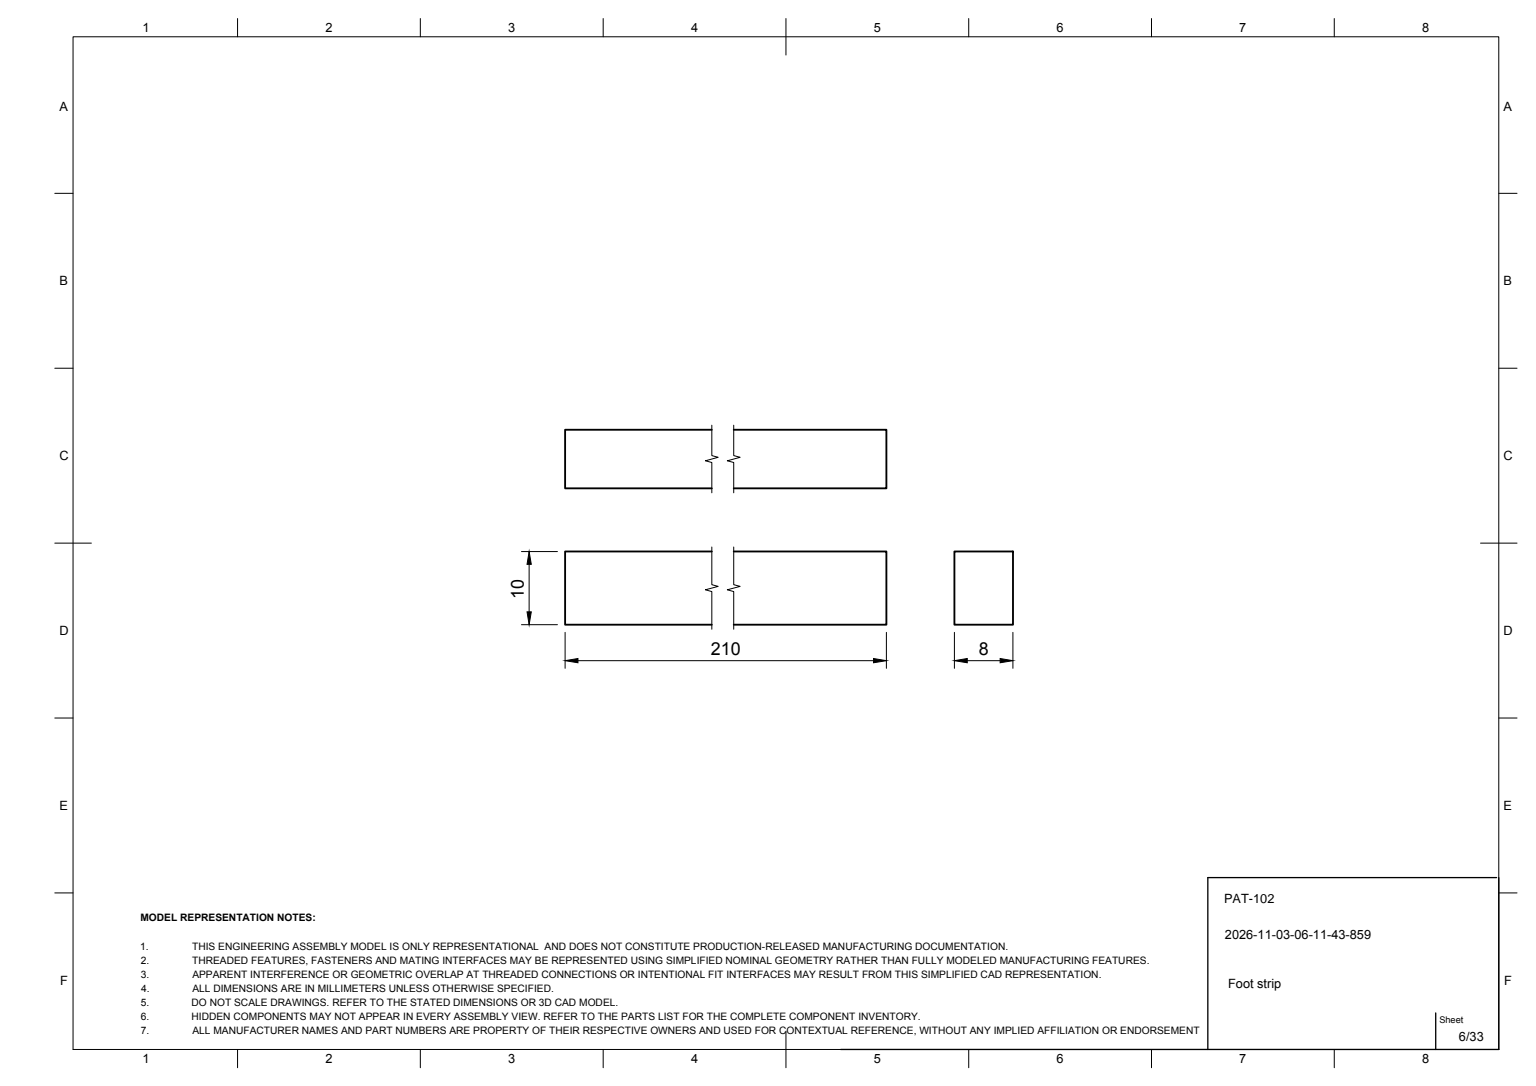
ISO-10303-21;
HEADER;
/* Generated by software containing ST-Developer
 * from STEP Tools, Inc. (www.steptools.com) 
 */

FILE_DESCRIPTION(
/* description */ ('Swing-away clamp arm'),
/* implementation_level */ '2;1');

FILE_NAME(
/* name */ 'Foot strip.step',
/* time_stamp */ '2026-10-28T03:26:03-07:00',
/* author */ (''),
/* organization */ (''),
/* preprocessor_version */ 'ST-DEVELOPER v20.2',
/* originating_system */ 'Autodesk Translation Framework v15.17.0.0',
/* authorisation */ '');

FILE_SCHEMA (('AUTOMOTIVE_DESIGN { 1 0 10303 214 3 1 1 }'));
ENDSEC;

DATA;
#10=MECHANICAL_DESIGN_GEOMETRIC_PRESENTATION_REPRESENTATION('',(#294),#10627);
#242=SHAPE_REPRESENTATION_RELATIONSHIP('SRR','None',#10740,#268);
#268=ADVANCED_BREP_SHAPE_REPRESENTATION('',(#328),#10599);
#294=STYLED_ITEM('',(#10951),#328);
#328=MANIFOLD_SOLID_BREP('Body1',#4900);
#464=PLANE('',#5245);
#465=PLANE('',#5246);
#466=PLANE('',#5247);
#467=PLANE('',#5248);
#468=PLANE('',#5249);
#469=PLANE('',#5250);
#647=FACE_OUTER_BOUND('',#962,.T.);
#648=FACE_OUTER_BOUND('',#963,.T.);
#649=FACE_OUTER_BOUND('',#964,.T.);
#650=FACE_OUTER_BOUND('',#965,.T.);
#651=FACE_OUTER_BOUND('',#966,.T.);
#652=FACE_OUTER_BOUND('',#967,.T.);
#962=EDGE_LOOP('',(#3329,#3330,#3331,#3332));
#963=EDGE_LOOP('',(#3333,#3334,#3335,#3336));
#964=EDGE_LOOP('',(#3337,#3338,#3339,#3340));
#965=EDGE_LOOP('',(#3341,#3342,#3343,#3344));
#966=EDGE_LOOP('',(#3345,#3346,#3347,#3348));
#967=EDGE_LOOP('',(#3349,#3350,#3351,#3352));
#1367=LINE('',#7543,#1689);
#1368=LINE('',#7545,#1690);
#1369=LINE('',#7547,#1691);
#1370=LINE('',#7548,#1692);
#1371=LINE('',#7551,#1693);
#1372=LINE('',#7553,#1694);
#1373=LINE('',#7554,#1695);
#1374=LINE('',#7557,#1696);
#1375=LINE('',#7559,#1697);
#1376=LINE('',#7560,#1698);
#1377=LINE('',#7562,#1699);
#1378=LINE('',#7563,#1700);
#1689=VECTOR('',#5932,1.);
#1690=VECTOR('',#5933,1.);
#1691=VECTOR('',#5934,1.);
#1692=VECTOR('',#5935,1.);
#1693=VECTOR('',#5938,1.);
#1694=VECTOR('',#5939,1.);
#1695=VECTOR('',#5940,1.);
#1696=VECTOR('',#5943,1.);
#1697=VECTOR('',#5944,1.);
#1698=VECTOR('',#5945,1.);
#1699=VECTOR('',#5948,1.);
#1700=VECTOR('',#5949,1.);
#2278=VERTEX_POINT('',#7541);
#2279=VERTEX_POINT('',#7542);
#2280=VERTEX_POINT('',#7544);
#2281=VERTEX_POINT('',#7546);
#2282=VERTEX_POINT('',#7550);
#2283=VERTEX_POINT('',#7552);
#2284=VERTEX_POINT('',#7556);
#2285=VERTEX_POINT('',#7558);
#2697=EDGE_CURVE('',#2278,#2279,#1367,.T.);
#2698=EDGE_CURVE('',#2279,#2280,#1368,.T.);
#2699=EDGE_CURVE('',#2281,#2280,#1369,.T.);
#2700=EDGE_CURVE('',#2278,#2281,#1370,.T.);
#2701=EDGE_CURVE('',#2282,#2278,#1371,.T.);
#2702=EDGE_CURVE('',#2283,#2281,#1372,.T.);
#2703=EDGE_CURVE('',#2282,#2283,#1373,.T.);
#2704=EDGE_CURVE('',#2284,#2282,#1374,.T.);
#2705=EDGE_CURVE('',#2285,#2283,#1375,.T.);
#2706=EDGE_CURVE('',#2284,#2285,#1376,.T.);
#2707=EDGE_CURVE('',#2279,#2284,#1377,.T.);
#2708=EDGE_CURVE('',#2280,#2285,#1378,.T.);
#3329=ORIENTED_EDGE('',*,*,#2697,.T.);
#3330=ORIENTED_EDGE('',*,*,#2698,.T.);
#3331=ORIENTED_EDGE('',*,*,#2699,.F.);
#3332=ORIENTED_EDGE('',*,*,#2700,.F.);
#3333=ORIENTED_EDGE('',*,*,#2701,.T.);
#3334=ORIENTED_EDGE('',*,*,#2700,.T.);
#3335=ORIENTED_EDGE('',*,*,#2702,.F.);
#3336=ORIENTED_EDGE('',*,*,#2703,.F.);
#3337=ORIENTED_EDGE('',*,*,#2704,.T.);
#3338=ORIENTED_EDGE('',*,*,#2703,.T.);
#3339=ORIENTED_EDGE('',*,*,#2705,.F.);
#3340=ORIENTED_EDGE('',*,*,#2706,.F.);
#3341=ORIENTED_EDGE('',*,*,#2707,.T.);
#3342=ORIENTED_EDGE('',*,*,#2706,.T.);
#3343=ORIENTED_EDGE('',*,*,#2708,.F.);
#3344=ORIENTED_EDGE('',*,*,#2698,.F.);
#3345=ORIENTED_EDGE('',*,*,#2708,.T.);
#3346=ORIENTED_EDGE('',*,*,#2705,.T.);
#3347=ORIENTED_EDGE('',*,*,#2702,.T.);
#3348=ORIENTED_EDGE('',*,*,#2699,.T.);
#3349=ORIENTED_EDGE('',*,*,#2707,.F.);
#3350=ORIENTED_EDGE('',*,*,#2697,.F.);
#3351=ORIENTED_EDGE('',*,*,#2701,.F.);
#3352=ORIENTED_EDGE('',*,*,#2704,.F.);
#4602=ADVANCED_FACE('',(#647),#464,.T.);
#4603=ADVANCED_FACE('',(#648),#465,.T.);
#4604=ADVANCED_FACE('',(#649),#466,.T.);
#4605=ADVANCED_FACE('',(#650),#467,.T.);
#4606=ADVANCED_FACE('',(#651),#468,.T.);
#4607=ADVANCED_FACE('',(#652),#469,.F.);
#4900=CLOSED_SHELL('',(#4602,#4603,#4604,#4605,#4606,#4607));
#5244=AXIS2_PLACEMENT_3D('',#7539,#5928,#5929);
#5245=AXIS2_PLACEMENT_3D('',#7540,#5930,#5931);
#5246=AXIS2_PLACEMENT_3D('',#7549,#5936,#5937);
#5247=AXIS2_PLACEMENT_3D('',#7555,#5941,#5942);
#5248=AXIS2_PLACEMENT_3D('',#7561,#5946,#5947);
#5249=AXIS2_PLACEMENT_3D('',#7564,#5950,#5951);
#5250=AXIS2_PLACEMENT_3D('',#7565,#5952,#5953);
#5928=DIRECTION('axis',(0.,0.,1.));
#5929=DIRECTION('refdir',(1.,0.,0.));
#5930=DIRECTION('center_axis',(0.,1.,0.));
#5931=DIRECTION('ref_axis',(-1.,0.,0.));
#5932=DIRECTION('',(-1.,0.,0.));
#5933=DIRECTION('',(0.,0.,1.));
#5934=DIRECTION('',(-1.,0.,0.));
#5935=DIRECTION('',(0.,0.,1.));
#5936=DIRECTION('center_axis',(1.,0.,0.));
#5937=DIRECTION('ref_axis',(0.,1.,0.));
#5938=DIRECTION('',(0.,1.,0.));
#5939=DIRECTION('',(0.,1.,0.));
#5940=DIRECTION('',(0.,0.,1.));
#5941=DIRECTION('center_axis',(0.,-1.,0.));
#5942=DIRECTION('ref_axis',(1.,0.,0.));
#5943=DIRECTION('',(1.,0.,0.));
#5944=DIRECTION('',(1.,0.,0.));
#5945=DIRECTION('',(0.,0.,1.));
#5946=DIRECTION('center_axis',(-1.,0.,0.));
#5947=DIRECTION('ref_axis',(0.,-1.,0.));
#5948=DIRECTION('',(0.,-1.,0.));
#5949=DIRECTION('',(0.,-1.,0.));
#5950=DIRECTION('center_axis',(0.,0.,1.));
#5951=DIRECTION('ref_axis',(1.,0.,0.));
#5952=DIRECTION('center_axis',(0.,0.,1.));
#5953=DIRECTION('ref_axis',(1.,0.,0.));
#7539=CARTESIAN_POINT('',(0.,0.,0.));
#7540=CARTESIAN_POINT('Origin',(-3.5,15.5,-0.8));
#7541=CARTESIAN_POINT('',(-3.5,15.5,-0.8));
#7542=CARTESIAN_POINT('',(-4.5,15.5,-0.8));
#7543=CARTESIAN_POINT('',(-3.5,15.5,-0.8));
#7544=CARTESIAN_POINT('',(-4.5,15.5,0.));
#7545=CARTESIAN_POINT('',(-4.5,15.5,-0.8));
#7546=CARTESIAN_POINT('',(-3.5,15.5,0.));
#7547=CARTESIAN_POINT('',(-3.5,15.5,0.));
#7548=CARTESIAN_POINT('',(-3.5,15.5,-0.8));
#7549=CARTESIAN_POINT('Origin',(-3.5,-5.5,-0.8));
#7550=CARTESIAN_POINT('',(-3.5,-5.5,-0.8));
#7551=CARTESIAN_POINT('',(-3.5,-5.5,-0.8));
#7552=CARTESIAN_POINT('',(-3.5,-5.5,0.));
#7553=CARTESIAN_POINT('',(-3.5,-5.5,0.));
#7554=CARTESIAN_POINT('',(-3.5,-5.5,-0.8));
#7555=CARTESIAN_POINT('Origin',(-4.5,-5.5,-0.8));
#7556=CARTESIAN_POINT('',(-4.5,-5.5,-0.8));
#7557=CARTESIAN_POINT('',(-4.5,-5.5,-0.8));
#7558=CARTESIAN_POINT('',(-4.5,-5.5,0.));
#7559=CARTESIAN_POINT('',(-4.5,-5.5,0.));
#7560=CARTESIAN_POINT('',(-4.5,-5.5,-0.8));
#7561=CARTESIAN_POINT('Origin',(-4.5,15.5,-0.8));
#7562=CARTESIAN_POINT('',(-4.5,15.5,-0.8));
#7563=CARTESIAN_POINT('',(-4.5,15.5,0.));
#7564=CARTESIAN_POINT('Origin',(-4.,5.,0.));
#7565=CARTESIAN_POINT('Origin',(-4.,5.,-0.8));
#10567=UNCERTAINTY_MEASURE_WITH_UNIT(LENGTH_MEASURE(0.001),#10628,
'DISTANCE_ACCURACY_VALUE',
'Maximum model space distance between geometric entities at asserted c
onnectivities');
#10595=UNCERTAINTY_MEASURE_WITH_UNIT(LENGTH_MEASURE(0.001),#10628,
'DISTANCE_ACCURACY_VALUE',
'Maximum model space distance between geometric entities at asserted c
onnectivities');
#10599=(
GEOMETRIC_REPRESENTATION_CONTEXT(3)
GLOBAL_UNCERTAINTY_ASSIGNED_CONTEXT((#10567))
GLOBAL_UNIT_ASSIGNED_CONTEXT((#10628,#10630,#10631))
REPRESENTATION_CONTEXT('','3D')
);
#10627=(
GEOMETRIC_REPRESENTATION_CONTEXT(3)
GLOBAL_UNCERTAINTY_ASSIGNED_CONTEXT((#10595))
GLOBAL_UNIT_ASSIGNED_CONTEXT((#10628,#10630,#10631))
REPRESENTATION_CONTEXT('','3D')
);
#10628=(
LENGTH_UNIT()
NAMED_UNIT(*)
SI_UNIT(.CENTI.,.METRE.)
);
#10630=(
NAMED_UNIT(*)
PLANE_ANGLE_UNIT()
SI_UNIT($,.RADIAN.)
);
#10631=(
NAMED_UNIT(*)
SI_UNIT($,.STERADIAN.)
SOLID_ANGLE_UNIT()
);
#10635=SHAPE_DEFINITION_REPRESENTATION(#10666,#10740);
#10666=PRODUCT_DEFINITION_SHAPE('',$,#10772);
#10740=SHAPE_REPRESENTATION('',(#5244),#10599);
#10768=PRODUCT_DEFINITION_CONTEXT('part definition',#10863,'design');
#10772=PRODUCT_DEFINITION('Foot strip','Foot strip',#10803,#10768);
#10803=PRODUCT_DEFINITION_FORMATION('',$,#10868);
#10863=APPLICATION_CONTEXT(
'Core Data for Automotive Mechanical Design Process');
#10864=PRODUCT_CONTEXT('part definition',#10863,'mechanical');
#10868=PRODUCT('Foot strip','Foot strip','Foot strip',(#10864));
#10945=COLOUR_RGB('Light Blue',0.38,0.62,0.78);
#10946=FILL_AREA_STYLE_COLOUR('',#10945);
#10947=FILL_AREA_STYLE('',(#10946));
#10948=SURFACE_STYLE_FILL_AREA(#10947);
#10949=SURFACE_SIDE_STYLE('',(#10948));
#10950=SURFACE_STYLE_USAGE(.BOTH.,#10949);
#10951=PRESENTATION_STYLE_ASSIGNMENT((#10950));
ENDSEC;
END-ISO-10303-21;
